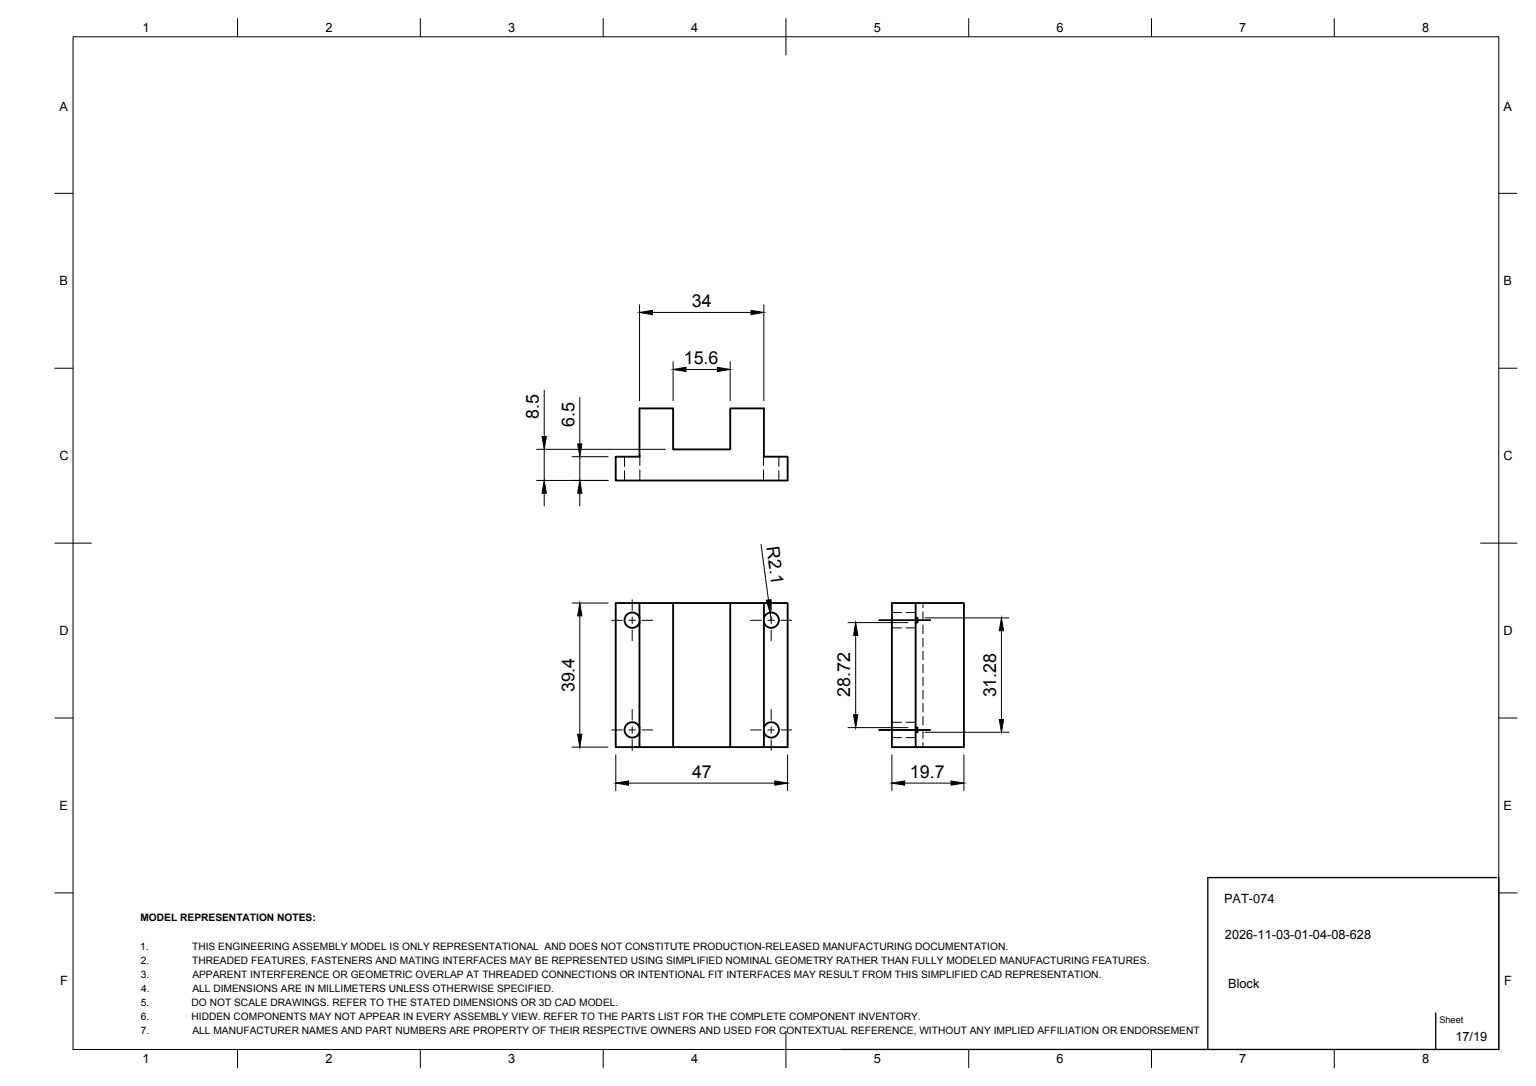
ISO-10303-21;
HEADER;
/* Generated by software containing ST-Developer
 * from STEP Tools, Inc. (www.steptools.com) 
 */

FILE_DESCRIPTION(
/* description */ ('Manual rail carriage with stops'),
/* implementation_level */ '2;1');

FILE_NAME(
/* name */ 'Block.step',
/* time_stamp */ '2026-10-27T18:54:27-07:00',
/* author */ (''),
/* organization */ (''),
/* preprocessor_version */ 'ST-DEVELOPER v20.2',
/* originating_system */ 'Autodesk Translation Framework v15.17.0.0',
/* authorisation */ '');

FILE_SCHEMA (('AUTOMOTIVE_DESIGN { 1 0 10303 214 3 1 1 }'));
ENDSEC;

DATA;
#10=MECHANICAL_DESIGN_GEOMETRIC_PRESENTATION_REPRESENTATION('',(#282),#8499);
#246=SHAPE_REPRESENTATION_RELATIONSHIP('SRR','None',#8611,#264);
#264=ADVANCED_BREP_SHAPE_REPRESENTATION('',(#298),#8490);
#282=STYLED_ITEM('',(#8767),#298);
#298=MANIFOLD_SOLID_BREP('Body1',#4952);
#356=FACE_BOUND('',#1071,.T.);
#357=FACE_BOUND('',#1072,.T.);
#358=FACE_BOUND('',#1073,.T.);
#359=FACE_BOUND('',#1074,.T.);
#505=PLANE('',#5415);
#506=PLANE('',#5421);
#507=PLANE('',#5427);
#508=PLANE('',#5433);
#509=PLANE('',#5439);
#510=PLANE('',#5440);
#511=PLANE('',#5441);
#512=PLANE('',#5442);
#513=PLANE('',#5443);
#514=PLANE('',#5444);
#515=PLANE('',#5445);
#516=PLANE('',#5446);
#517=PLANE('',#5447);
#518=PLANE('',#5448);
#519=PLANE('',#5449);
#520=PLANE('',#5450);
#521=PLANE('',#5451);
#522=PLANE('',#5452);
#741=FACE_OUTER_BOUND('',#1057,.T.);
#742=FACE_OUTER_BOUND('',#1058,.T.);
#743=FACE_OUTER_BOUND('',#1059,.T.);
#744=FACE_OUTER_BOUND('',#1060,.T.);
#745=FACE_OUTER_BOUND('',#1061,.T.);
#746=FACE_OUTER_BOUND('',#1062,.T.);
#747=FACE_OUTER_BOUND('',#1063,.T.);
#748=FACE_OUTER_BOUND('',#1064,.T.);
#749=FACE_OUTER_BOUND('',#1065,.T.);
#750=FACE_OUTER_BOUND('',#1066,.T.);
#751=FACE_OUTER_BOUND('',#1067,.T.);
#752=FACE_OUTER_BOUND('',#1068,.T.);
#753=FACE_OUTER_BOUND('',#1069,.T.);
#754=FACE_OUTER_BOUND('',#1070,.T.);
#755=FACE_OUTER_BOUND('',#1075,.T.);
#756=FACE_OUTER_BOUND('',#1076,.T.);
#757=FACE_OUTER_BOUND('',#1077,.T.);
#758=FACE_OUTER_BOUND('',#1078,.T.);
#759=FACE_OUTER_BOUND('',#1079,.T.);
#760=FACE_OUTER_BOUND('',#1080,.T.);
#761=FACE_OUTER_BOUND('',#1081,.T.);
#762=FACE_OUTER_BOUND('',#1082,.T.);
#1057=EDGE_LOOP('',(#4156,#4157));
#1058=EDGE_LOOP('',(#4158,#4159,#4160,#4161,#4162,#4163,#4164,#4165));
#1059=EDGE_LOOP('',(#4166,#4167));
#1060=EDGE_LOOP('',(#4168,#4169,#4170,#4171,#4172,#4173,#4174,#4175));
#1061=EDGE_LOOP('',(#4176,#4177));
#1062=EDGE_LOOP('',(#4178,#4179,#4180,#4181,#4182,#4183,#4184,#4185));
#1063=EDGE_LOOP('',(#4186,#4187));
#1064=EDGE_LOOP('',(#4188,#4189,#4190,#4191,#4192,#4193,#4194,#4195));
#1065=EDGE_LOOP('',(#4196,#4197,#4198,#4199,#4200,#4201,#4202,#4203,#4204,
#4205,#4206,#4207));
#1066=EDGE_LOOP('',(#4208,#4209,#4210,#4211,#4212,#4213,#4214,#4215,#4216,
#4217,#4218,#4219));
#1067=EDGE_LOOP('',(#4220,#4221,#4222,#4223,#4224,#4225,#4226,#4227,#4228,
#4229,#4230,#4231));
#1068=EDGE_LOOP('',(#4232,#4233,#4234,#4235,#4236,#4237,#4238,#4239,#4240,
#4241));
#1069=EDGE_LOOP('',(#4242,#4243,#4244,#4245));
#1070=EDGE_LOOP('',(#4246,#4247,#4248,#4249));
#1071=EDGE_LOOP('',(#4250));
#1072=EDGE_LOOP('',(#4251));
#1073=EDGE_LOOP('',(#4252));
#1074=EDGE_LOOP('',(#4253));
#1075=EDGE_LOOP('',(#4254,#4255,#4256,#4257));
#1076=EDGE_LOOP('',(#4258,#4259,#4260,#4261,#4262,#4263,#4264,#4265,#4266,
#4267));
#1077=EDGE_LOOP('',(#4268,#4269,#4270,#4271));
#1078=EDGE_LOOP('',(#4272,#4273,#4274,#4275));
#1079=EDGE_LOOP('',(#4276,#4277,#4278,#4279));
#1080=EDGE_LOOP('',(#4280,#4281,#4282,#4283));
#1081=EDGE_LOOP('',(#4284,#4285,#4286,#4287));
#1082=EDGE_LOOP('',(#4288,#4289,#4290,#4291,#4292,#4293,#4294,#4295,#4296,
#4297,#4298,#4299));
#1505=LINE('',#7911,#2005);
#1506=LINE('',#7915,#2006);
#1507=LINE('',#7919,#2007);
#1508=LINE('',#7923,#2008);
#1509=LINE('',#7927,#2009);
#1510=LINE('',#7931,#2010);
#1511=LINE('',#7935,#2011);
#1512=LINE('',#7939,#2012);
#1513=LINE('',#7943,#2013);
#1514=LINE('',#7947,#2014);
#1515=LINE('',#7951,#2015);
#1516=LINE('',#7955,#2016);
#1517=LINE('',#7959,#2017);
#1518=LINE('',#7963,#2018);
#1519=LINE('',#7967,#2019);
#1520=LINE('',#7971,#2020);
#1521=LINE('',#7973,#2021);
#1522=LINE('',#7975,#2022);
#1523=LINE('',#7977,#2023);
#1524=LINE('',#7979,#2024);
#1525=LINE('',#7981,#2025);
#1526=LINE('',#7982,#2026);
#1527=LINE('',#7984,#2027);
#1528=LINE('',#7986,#2028);
#1529=LINE('',#7988,#2029);
#1530=LINE('',#7990,#2030);
#1531=LINE('',#7992,#2031);
#1532=LINE('',#7993,#2032);
#1533=LINE('',#7996,#2033);
#1534=LINE('',#7998,#2034);
#1535=LINE('',#8000,#2035);
#1536=LINE('',#8002,#2036);
#1537=LINE('',#8003,#2037);
#1538=LINE('',#8005,#2038);
#1539=LINE('',#8007,#2039);
#1540=LINE('',#8009,#2040);
#1541=LINE('',#8011,#2041);
#1542=LINE('',#8012,#2042);
#1543=LINE('',#8015,#2043);
#1544=LINE('',#8016,#2044);
#1545=LINE('',#8019,#2045);
#1546=LINE('',#8020,#2046);
#1547=LINE('',#8023,#2047);
#1548=LINE('',#8024,#2048);
#1549=LINE('',#8027,#2049);
#1550=LINE('',#8028,#2050);
#1551=LINE('',#8030,#2051);
#1552=LINE('',#8033,#2052);
#1553=LINE('',#8034,#2053);
#1554=LINE('',#8037,#2054);
#1555=LINE('',#8038,#2055);
#1556=LINE('',#8041,#2056);
#1557=LINE('',#8042,#2057);
#1558=LINE('',#8045,#2058);
#1559=LINE('',#8046,#2059);
#1560=LINE('',#8048,#2060);
#2005=VECTOR('',#6462,1.);
#2006=VECTOR('',#6467,1.);
#2007=VECTOR('',#6470,0.21);
#2008=VECTOR('',#6475,1.);
#2009=VECTOR('',#6478,1.);
#2010=VECTOR('',#6483,1.);
#2011=VECTOR('',#6486,0.21);
#2012=VECTOR('',#6491,1.);
#2013=VECTOR('',#6494,1.);
#2014=VECTOR('',#6499,1.);
#2015=VECTOR('',#6502,0.21);
#2016=VECTOR('',#6507,1.);
#2017=VECTOR('',#6510,1.);
#2018=VECTOR('',#6515,1.);
#2019=VECTOR('',#6518,0.21);
#2020=VECTOR('',#6523,1.);
#2021=VECTOR('',#6526,1.);
#2022=VECTOR('',#6527,1.);
#2023=VECTOR('',#6528,1.);
#2024=VECTOR('',#6529,1.);
#2025=VECTOR('',#6530,1.);
#2026=VECTOR('',#6531,1.);
#2027=VECTOR('',#6534,1.);
#2028=VECTOR('',#6535,1.);
#2029=VECTOR('',#6536,1.);
#2030=VECTOR('',#6537,1.);
#2031=VECTOR('',#6538,1.);
#2032=VECTOR('',#6539,1.);
#2033=VECTOR('',#6542,1.);
#2034=VECTOR('',#6543,1.);
#2035=VECTOR('',#6544,1.);
#2036=VECTOR('',#6545,1.);
#2037=VECTOR('',#6546,1.);
#2038=VECTOR('',#6547,1.);
#2039=VECTOR('',#6548,1.);
#2040=VECTOR('',#6549,1.);
#2041=VECTOR('',#6550,1.);
#2042=VECTOR('',#6551,1.);
#2043=VECTOR('',#6554,1.);
#2044=VECTOR('',#6555,1.);
#2045=VECTOR('',#6558,1.);
#2046=VECTOR('',#6559,1.);
#2047=VECTOR('',#6562,1.);
#2048=VECTOR('',#6563,1.);
#2049=VECTOR('',#6566,1.);
#2050=VECTOR('',#6567,1.);
#2051=VECTOR('',#6570,1.);
#2052=VECTOR('',#6573,1.);
#2053=VECTOR('',#6574,1.);
#2054=VECTOR('',#6577,1.);
#2055=VECTOR('',#6578,1.);
#2056=VECTOR('',#6581,1.);
#2057=VECTOR('',#6582,1.);
#2058=VECTOR('',#6585,1.);
#2059=VECTOR('',#6586,1.);
#2060=VECTOR('',#6589,1.);
#2255=CIRCLE('',#5416,0.21);
#2256=CIRCLE('',#5418,0.21);
#2257=CIRCLE('',#5419,0.21);
#2258=CIRCLE('',#5420,0.21);
#2259=CIRCLE('',#5422,0.21);
#2260=CIRCLE('',#5424,0.21);
#2261=CIRCLE('',#5425,0.21);
#2262=CIRCLE('',#5426,0.21);
#2263=CIRCLE('',#5428,0.21);
#2264=CIRCLE('',#5430,0.21);
#2265=CIRCLE('',#5431,0.21);
#2266=CIRCLE('',#5432,0.21);
#2267=CIRCLE('',#5434,0.21);
#2268=CIRCLE('',#5436,0.21);
#2269=CIRCLE('',#5437,0.21);
#2270=CIRCLE('',#5438,0.21);
#2575=VERTEX_POINT('',#7909);
#2576=VERTEX_POINT('',#7910);
#2577=VERTEX_POINT('',#7914);
#2578=VERTEX_POINT('',#7916);
#2579=VERTEX_POINT('',#7918);
#2580=VERTEX_POINT('',#7921);
#2581=VERTEX_POINT('',#7925);
#2582=VERTEX_POINT('',#7926);
#2583=VERTEX_POINT('',#7930);
#2584=VERTEX_POINT('',#7932);
#2585=VERTEX_POINT('',#7934);
#2586=VERTEX_POINT('',#7937);
#2587=VERTEX_POINT('',#7941);
#2588=VERTEX_POINT('',#7942);
#2589=VERTEX_POINT('',#7946);
#2590=VERTEX_POINT('',#7948);
#2591=VERTEX_POINT('',#7950);
#2592=VERTEX_POINT('',#7953);
#2593=VERTEX_POINT('',#7957);
#2594=VERTEX_POINT('',#7958);
#2595=VERTEX_POINT('',#7962);
#2596=VERTEX_POINT('',#7964);
#2597=VERTEX_POINT('',#7966);
#2598=VERTEX_POINT('',#7969);
#2599=VERTEX_POINT('',#7974);
#2600=VERTEX_POINT('',#7976);
#2601=VERTEX_POINT('',#7978);
#2602=VERTEX_POINT('',#7980);
#2603=VERTEX_POINT('',#7985);
#2604=VERTEX_POINT('',#7987);
#2605=VERTEX_POINT('',#7989);
#2606=VERTEX_POINT('',#7991);
#2607=VERTEX_POINT('',#7995);
#2608=VERTEX_POINT('',#7997);
#2609=VERTEX_POINT('',#7999);
#2610=VERTEX_POINT('',#8001);
#2611=VERTEX_POINT('',#8004);
#2612=VERTEX_POINT('',#8006);
#2613=VERTEX_POINT('',#8008);
#2614=VERTEX_POINT('',#8010);
#2615=VERTEX_POINT('',#8014);
#2616=VERTEX_POINT('',#8018);
#2617=VERTEX_POINT('',#8022);
#2618=VERTEX_POINT('',#8026);
#2619=VERTEX_POINT('',#8032);
#2620=VERTEX_POINT('',#8036);
#2621=VERTEX_POINT('',#8040);
#2622=VERTEX_POINT('',#8044);
#3126=EDGE_CURVE('',#2575,#2576,#1505,.T.);
#3127=EDGE_CURVE('',#2575,#2576,#2255,.T.);
#3128=EDGE_CURVE('',#2577,#2575,#1506,.T.);
#3129=EDGE_CURVE('',#2578,#2577,#2256,.T.);
#3130=EDGE_CURVE('',#2578,#2579,#1507,.T.);
#3131=EDGE_CURVE('',#2579,#2579,#2257,.T.);
#3132=EDGE_CURVE('',#2580,#2578,#2258,.T.);
#3133=EDGE_CURVE('',#2576,#2580,#1508,.T.);
#3134=EDGE_CURVE('',#2581,#2582,#1509,.T.);
#3135=EDGE_CURVE('',#2581,#2582,#2259,.T.);
#3136=EDGE_CURVE('',#2583,#2581,#1510,.T.);
#3137=EDGE_CURVE('',#2584,#2583,#2260,.T.);
#3138=EDGE_CURVE('',#2584,#2585,#1511,.T.);
#3139=EDGE_CURVE('',#2585,#2585,#2261,.T.);
#3140=EDGE_CURVE('',#2586,#2584,#2262,.T.);
#3141=EDGE_CURVE('',#2582,#2586,#1512,.T.);
#3142=EDGE_CURVE('',#2587,#2588,#1513,.T.);
#3143=EDGE_CURVE('',#2587,#2588,#2263,.T.);
#3144=EDGE_CURVE('',#2589,#2587,#1514,.T.);
#3145=EDGE_CURVE('',#2590,#2589,#2264,.T.);
#3146=EDGE_CURVE('',#2590,#2591,#1515,.T.);
#3147=EDGE_CURVE('',#2591,#2591,#2265,.T.);
#3148=EDGE_CURVE('',#2592,#2590,#2266,.T.);
#3149=EDGE_CURVE('',#2588,#2592,#1516,.T.);
#3150=EDGE_CURVE('',#2593,#2594,#1517,.T.);
#3151=EDGE_CURVE('',#2593,#2594,#2267,.T.);
#3152=EDGE_CURVE('',#2595,#2593,#1518,.T.);
#3153=EDGE_CURVE('',#2596,#2595,#2268,.T.);
#3154=EDGE_CURVE('',#2596,#2597,#1519,.T.);
#3155=EDGE_CURVE('',#2597,#2597,#2269,.T.);
#3156=EDGE_CURVE('',#2598,#2596,#2270,.T.);
#3157=EDGE_CURVE('',#2594,#2598,#1520,.T.);
#3158=EDGE_CURVE('',#2580,#2589,#1521,.T.);
#3159=EDGE_CURVE('',#2592,#2599,#1522,.T.);
#3160=EDGE_CURVE('',#2600,#2599,#1523,.T.);
#3161=EDGE_CURVE('',#2600,#2601,#1524,.T.);
#3162=EDGE_CURVE('',#2602,#2601,#1525,.T.);
#3163=EDGE_CURVE('',#2602,#2577,#1526,.T.);
#3164=EDGE_CURVE('',#2586,#2595,#1527,.T.);
#3165=EDGE_CURVE('',#2598,#2603,#1528,.T.);
#3166=EDGE_CURVE('',#2604,#2603,#1529,.T.);
#3167=EDGE_CURVE('',#2605,#2604,#1530,.T.);
#3168=EDGE_CURVE('',#2606,#2605,#1531,.T.);
#3169=EDGE_CURVE('',#2606,#2583,#1532,.T.);
#3170=EDGE_CURVE('',#2599,#2607,#1533,.T.);
#3171=EDGE_CURVE('',#2607,#2608,#1534,.T.);
#3172=EDGE_CURVE('',#2608,#2609,#1535,.T.);
#3173=EDGE_CURVE('',#2609,#2610,#1536,.T.);
#3174=EDGE_CURVE('',#2610,#2606,#1537,.T.);
#3175=EDGE_CURVE('',#2605,#2611,#1538,.T.);
#3176=EDGE_CURVE('',#2611,#2612,#1539,.T.);
#3177=EDGE_CURVE('',#2612,#2613,#1540,.T.);
#3178=EDGE_CURVE('',#2613,#2614,#1541,.T.);
#3179=EDGE_CURVE('',#2614,#2600,#1542,.T.);
#3180=EDGE_CURVE('',#2615,#2602,#1543,.T.);
#3181=EDGE_CURVE('',#2607,#2615,#1544,.T.);
#3182=EDGE_CURVE('',#2616,#2615,#1545,.T.);
#3183=EDGE_CURVE('',#2608,#2616,#1546,.T.);
#3184=EDGE_CURVE('',#2617,#2616,#1547,.T.);
#3185=EDGE_CURVE('',#2609,#2617,#1548,.T.);
#3186=EDGE_CURVE('',#2618,#2617,#1549,.T.);
#3187=EDGE_CURVE('',#2610,#2618,#1550,.T.);
#3188=EDGE_CURVE('',#2603,#2618,#1551,.T.);
#3189=EDGE_CURVE('',#2619,#2604,#1552,.T.);
#3190=EDGE_CURVE('',#2611,#2619,#1553,.T.);
#3191=EDGE_CURVE('',#2620,#2619,#1554,.T.);
#3192=EDGE_CURVE('',#2612,#2620,#1555,.T.);
#3193=EDGE_CURVE('',#2621,#2620,#1556,.T.);
#3194=EDGE_CURVE('',#2613,#2621,#1557,.T.);
#3195=EDGE_CURVE('',#2622,#2621,#1558,.T.);
#3196=EDGE_CURVE('',#2614,#2622,#1559,.T.);
#3197=EDGE_CURVE('',#2601,#2622,#1560,.T.);
#4156=ORIENTED_EDGE('',*,*,#3126,.F.);
#4157=ORIENTED_EDGE('',*,*,#3127,.T.);
#4158=ORIENTED_EDGE('',*,*,#3128,.F.);
#4159=ORIENTED_EDGE('',*,*,#3129,.F.);
#4160=ORIENTED_EDGE('',*,*,#3130,.T.);
#4161=ORIENTED_EDGE('',*,*,#3131,.F.);
#4162=ORIENTED_EDGE('',*,*,#3130,.F.);
#4163=ORIENTED_EDGE('',*,*,#3132,.F.);
#4164=ORIENTED_EDGE('',*,*,#3133,.F.);
#4165=ORIENTED_EDGE('',*,*,#3127,.F.);
#4166=ORIENTED_EDGE('',*,*,#3134,.F.);
#4167=ORIENTED_EDGE('',*,*,#3135,.T.);
#4168=ORIENTED_EDGE('',*,*,#3136,.F.);
#4169=ORIENTED_EDGE('',*,*,#3137,.F.);
#4170=ORIENTED_EDGE('',*,*,#3138,.T.);
#4171=ORIENTED_EDGE('',*,*,#3139,.F.);
#4172=ORIENTED_EDGE('',*,*,#3138,.F.);
#4173=ORIENTED_EDGE('',*,*,#3140,.F.);
#4174=ORIENTED_EDGE('',*,*,#3141,.F.);
#4175=ORIENTED_EDGE('',*,*,#3135,.F.);
#4176=ORIENTED_EDGE('',*,*,#3142,.F.);
#4177=ORIENTED_EDGE('',*,*,#3143,.T.);
#4178=ORIENTED_EDGE('',*,*,#3144,.F.);
#4179=ORIENTED_EDGE('',*,*,#3145,.F.);
#4180=ORIENTED_EDGE('',*,*,#3146,.T.);
#4181=ORIENTED_EDGE('',*,*,#3147,.F.);
#4182=ORIENTED_EDGE('',*,*,#3146,.F.);
#4183=ORIENTED_EDGE('',*,*,#3148,.F.);
#4184=ORIENTED_EDGE('',*,*,#3149,.F.);
#4185=ORIENTED_EDGE('',*,*,#3143,.F.);
#4186=ORIENTED_EDGE('',*,*,#3150,.F.);
#4187=ORIENTED_EDGE('',*,*,#3151,.T.);
#4188=ORIENTED_EDGE('',*,*,#3152,.F.);
#4189=ORIENTED_EDGE('',*,*,#3153,.F.);
#4190=ORIENTED_EDGE('',*,*,#3154,.T.);
#4191=ORIENTED_EDGE('',*,*,#3155,.F.);
#4192=ORIENTED_EDGE('',*,*,#3154,.F.);
#4193=ORIENTED_EDGE('',*,*,#3156,.F.);
#4194=ORIENTED_EDGE('',*,*,#3157,.F.);
#4195=ORIENTED_EDGE('',*,*,#3151,.F.);
#4196=ORIENTED_EDGE('',*,*,#3128,.T.);
#4197=ORIENTED_EDGE('',*,*,#3126,.T.);
#4198=ORIENTED_EDGE('',*,*,#3133,.T.);
#4199=ORIENTED_EDGE('',*,*,#3158,.T.);
#4200=ORIENTED_EDGE('',*,*,#3144,.T.);
#4201=ORIENTED_EDGE('',*,*,#3142,.T.);
#4202=ORIENTED_EDGE('',*,*,#3149,.T.);
#4203=ORIENTED_EDGE('',*,*,#3159,.T.);
#4204=ORIENTED_EDGE('',*,*,#3160,.F.);
#4205=ORIENTED_EDGE('',*,*,#3161,.T.);
#4206=ORIENTED_EDGE('',*,*,#3162,.F.);
#4207=ORIENTED_EDGE('',*,*,#3163,.T.);
#4208=ORIENTED_EDGE('',*,*,#3136,.T.);
#4209=ORIENTED_EDGE('',*,*,#3134,.T.);
#4210=ORIENTED_EDGE('',*,*,#3141,.T.);
#4211=ORIENTED_EDGE('',*,*,#3164,.T.);
#4212=ORIENTED_EDGE('',*,*,#3152,.T.);
#4213=ORIENTED_EDGE('',*,*,#3150,.T.);
#4214=ORIENTED_EDGE('',*,*,#3157,.T.);
#4215=ORIENTED_EDGE('',*,*,#3165,.T.);
#4216=ORIENTED_EDGE('',*,*,#3166,.F.);
#4217=ORIENTED_EDGE('',*,*,#3167,.F.);
#4218=ORIENTED_EDGE('',*,*,#3168,.F.);
#4219=ORIENTED_EDGE('',*,*,#3169,.T.);
#4220=ORIENTED_EDGE('',*,*,#3160,.T.);
#4221=ORIENTED_EDGE('',*,*,#3170,.T.);
#4222=ORIENTED_EDGE('',*,*,#3171,.T.);
#4223=ORIENTED_EDGE('',*,*,#3172,.T.);
#4224=ORIENTED_EDGE('',*,*,#3173,.T.);
#4225=ORIENTED_EDGE('',*,*,#3174,.T.);
#4226=ORIENTED_EDGE('',*,*,#3168,.T.);
#4227=ORIENTED_EDGE('',*,*,#3175,.T.);
#4228=ORIENTED_EDGE('',*,*,#3176,.T.);
#4229=ORIENTED_EDGE('',*,*,#3177,.T.);
#4230=ORIENTED_EDGE('',*,*,#3178,.T.);
#4231=ORIENTED_EDGE('',*,*,#3179,.T.);
#4232=ORIENTED_EDGE('',*,*,#3132,.T.);
#4233=ORIENTED_EDGE('',*,*,#3129,.T.);
#4234=ORIENTED_EDGE('',*,*,#3163,.F.);
#4235=ORIENTED_EDGE('',*,*,#3180,.F.);
#4236=ORIENTED_EDGE('',*,*,#3181,.F.);
#4237=ORIENTED_EDGE('',*,*,#3170,.F.);
#4238=ORIENTED_EDGE('',*,*,#3159,.F.);
#4239=ORIENTED_EDGE('',*,*,#3148,.T.);
#4240=ORIENTED_EDGE('',*,*,#3145,.T.);
#4241=ORIENTED_EDGE('',*,*,#3158,.F.);
#4242=ORIENTED_EDGE('',*,*,#3181,.T.);
#4243=ORIENTED_EDGE('',*,*,#3182,.F.);
#4244=ORIENTED_EDGE('',*,*,#3183,.F.);
#4245=ORIENTED_EDGE('',*,*,#3171,.F.);
#4246=ORIENTED_EDGE('',*,*,#3183,.T.);
#4247=ORIENTED_EDGE('',*,*,#3184,.F.);
#4248=ORIENTED_EDGE('',*,*,#3185,.F.);
#4249=ORIENTED_EDGE('',*,*,#3172,.F.);
#4250=ORIENTED_EDGE('',*,*,#3131,.T.);
#4251=ORIENTED_EDGE('',*,*,#3139,.T.);
#4252=ORIENTED_EDGE('',*,*,#3147,.T.);
#4253=ORIENTED_EDGE('',*,*,#3155,.T.);
#4254=ORIENTED_EDGE('',*,*,#3185,.T.);
#4255=ORIENTED_EDGE('',*,*,#3186,.F.);
#4256=ORIENTED_EDGE('',*,*,#3187,.F.);
#4257=ORIENTED_EDGE('',*,*,#3173,.F.);
#4258=ORIENTED_EDGE('',*,*,#3140,.T.);
#4259=ORIENTED_EDGE('',*,*,#3137,.T.);
#4260=ORIENTED_EDGE('',*,*,#3169,.F.);
#4261=ORIENTED_EDGE('',*,*,#3174,.F.);
#4262=ORIENTED_EDGE('',*,*,#3187,.T.);
#4263=ORIENTED_EDGE('',*,*,#3188,.F.);
#4264=ORIENTED_EDGE('',*,*,#3165,.F.);
#4265=ORIENTED_EDGE('',*,*,#3156,.T.);
#4266=ORIENTED_EDGE('',*,*,#3153,.T.);
#4267=ORIENTED_EDGE('',*,*,#3164,.F.);
#4268=ORIENTED_EDGE('',*,*,#3167,.T.);
#4269=ORIENTED_EDGE('',*,*,#3189,.F.);
#4270=ORIENTED_EDGE('',*,*,#3190,.F.);
#4271=ORIENTED_EDGE('',*,*,#3175,.F.);
#4272=ORIENTED_EDGE('',*,*,#3190,.T.);
#4273=ORIENTED_EDGE('',*,*,#3191,.F.);
#4274=ORIENTED_EDGE('',*,*,#3192,.F.);
#4275=ORIENTED_EDGE('',*,*,#3176,.F.);
#4276=ORIENTED_EDGE('',*,*,#3192,.T.);
#4277=ORIENTED_EDGE('',*,*,#3193,.F.);
#4278=ORIENTED_EDGE('',*,*,#3194,.F.);
#4279=ORIENTED_EDGE('',*,*,#3177,.F.);
#4280=ORIENTED_EDGE('',*,*,#3194,.T.);
#4281=ORIENTED_EDGE('',*,*,#3195,.F.);
#4282=ORIENTED_EDGE('',*,*,#3196,.F.);
#4283=ORIENTED_EDGE('',*,*,#3178,.F.);
#4284=ORIENTED_EDGE('',*,*,#3196,.T.);
#4285=ORIENTED_EDGE('',*,*,#3197,.F.);
#4286=ORIENTED_EDGE('',*,*,#3161,.F.);
#4287=ORIENTED_EDGE('',*,*,#3179,.F.);
#4288=ORIENTED_EDGE('',*,*,#3162,.T.);
#4289=ORIENTED_EDGE('',*,*,#3197,.T.);
#4290=ORIENTED_EDGE('',*,*,#3195,.T.);
#4291=ORIENTED_EDGE('',*,*,#3193,.T.);
#4292=ORIENTED_EDGE('',*,*,#3191,.T.);
#4293=ORIENTED_EDGE('',*,*,#3189,.T.);
#4294=ORIENTED_EDGE('',*,*,#3166,.T.);
#4295=ORIENTED_EDGE('',*,*,#3188,.T.);
#4296=ORIENTED_EDGE('',*,*,#3186,.T.);
#4297=ORIENTED_EDGE('',*,*,#3184,.T.);
#4298=ORIENTED_EDGE('',*,*,#3182,.T.);
#4299=ORIENTED_EDGE('',*,*,#3180,.T.);
#4656=CYLINDRICAL_SURFACE('',#5417,0.21);
#4657=CYLINDRICAL_SURFACE('',#5423,0.21);
#4658=CYLINDRICAL_SURFACE('',#5429,0.21);
#4659=CYLINDRICAL_SURFACE('',#5435,0.21);
#4840=ADVANCED_FACE('',(#741),#505,.T.);
#4841=ADVANCED_FACE('',(#742),#4656,.F.);
#4842=ADVANCED_FACE('',(#743),#506,.T.);
#4843=ADVANCED_FACE('',(#744),#4657,.F.);
#4844=ADVANCED_FACE('',(#745),#507,.T.);
#4845=ADVANCED_FACE('',(#746),#4658,.F.);
#4846=ADVANCED_FACE('',(#747),#508,.T.);
#4847=ADVANCED_FACE('',(#748),#4659,.F.);
#4848=ADVANCED_FACE('',(#749),#509,.T.);
#4849=ADVANCED_FACE('',(#750),#510,.T.);
#4850=ADVANCED_FACE('',(#751),#511,.T.);
#4851=ADVANCED_FACE('',(#752),#512,.T.);
#4852=ADVANCED_FACE('',(#753),#513,.T.);
#4853=ADVANCED_FACE('',(#754,#356,#357,#358,#359),#514,.T.);
#4854=ADVANCED_FACE('',(#755),#515,.T.);
#4855=ADVANCED_FACE('',(#756),#516,.T.);
#4856=ADVANCED_FACE('',(#757),#517,.T.);
#4857=ADVANCED_FACE('',(#758),#518,.T.);
#4858=ADVANCED_FACE('',(#759),#519,.T.);
#4859=ADVANCED_FACE('',(#760),#520,.T.);
#4860=ADVANCED_FACE('',(#761),#521,.T.);
#4861=ADVANCED_FACE('',(#762),#522,.T.);
#4952=CLOSED_SHELL('',(#4840,#4841,#4842,#4843,#4844,#4845,#4846,#4847,
#4848,#4849,#4850,#4851,#4852,#4853,#4854,#4855,#4856,#4857,#4858,#4859,
#4860,#4861));
#5414=AXIS2_PLACEMENT_3D('',#7907,#6458,#6459);
#5415=AXIS2_PLACEMENT_3D('',#7908,#6460,#6461);
#5416=AXIS2_PLACEMENT_3D('',#7912,#6463,#6464);
#5417=AXIS2_PLACEMENT_3D('',#7913,#6465,#6466);
#5418=AXIS2_PLACEMENT_3D('',#7917,#6468,#6469);
#5419=AXIS2_PLACEMENT_3D('',#7920,#6471,#6472);
#5420=AXIS2_PLACEMENT_3D('',#7922,#6473,#6474);
#5421=AXIS2_PLACEMENT_3D('',#7924,#6476,#6477);
#5422=AXIS2_PLACEMENT_3D('',#7928,#6479,#6480);
#5423=AXIS2_PLACEMENT_3D('',#7929,#6481,#6482);
#5424=AXIS2_PLACEMENT_3D('',#7933,#6484,#6485);
#5425=AXIS2_PLACEMENT_3D('',#7936,#6487,#6488);
#5426=AXIS2_PLACEMENT_3D('',#7938,#6489,#6490);
#5427=AXIS2_PLACEMENT_3D('',#7940,#6492,#6493);
#5428=AXIS2_PLACEMENT_3D('',#7944,#6495,#6496);
#5429=AXIS2_PLACEMENT_3D('',#7945,#6497,#6498);
#5430=AXIS2_PLACEMENT_3D('',#7949,#6500,#6501);
#5431=AXIS2_PLACEMENT_3D('',#7952,#6503,#6504);
#5432=AXIS2_PLACEMENT_3D('',#7954,#6505,#6506);
#5433=AXIS2_PLACEMENT_3D('',#7956,#6508,#6509);
#5434=AXIS2_PLACEMENT_3D('',#7960,#6511,#6512);
#5435=AXIS2_PLACEMENT_3D('',#7961,#6513,#6514);
#5436=AXIS2_PLACEMENT_3D('',#7965,#6516,#6517);
#5437=AXIS2_PLACEMENT_3D('',#7968,#6519,#6520);
#5438=AXIS2_PLACEMENT_3D('',#7970,#6521,#6522);
#5439=AXIS2_PLACEMENT_3D('',#7972,#6524,#6525);
#5440=AXIS2_PLACEMENT_3D('',#7983,#6532,#6533);
#5441=AXIS2_PLACEMENT_3D('',#7994,#6540,#6541);
#5442=AXIS2_PLACEMENT_3D('',#8013,#6552,#6553);
#5443=AXIS2_PLACEMENT_3D('',#8017,#6556,#6557);
#5444=AXIS2_PLACEMENT_3D('',#8021,#6560,#6561);
#5445=AXIS2_PLACEMENT_3D('',#8025,#6564,#6565);
#5446=AXIS2_PLACEMENT_3D('',#8029,#6568,#6569);
#5447=AXIS2_PLACEMENT_3D('',#8031,#6571,#6572);
#5448=AXIS2_PLACEMENT_3D('',#8035,#6575,#6576);
#5449=AXIS2_PLACEMENT_3D('',#8039,#6579,#6580);
#5450=AXIS2_PLACEMENT_3D('',#8043,#6583,#6584);
#5451=AXIS2_PLACEMENT_3D('',#8047,#6587,#6588);
#5452=AXIS2_PLACEMENT_3D('',#8049,#6590,#6591);
#6458=DIRECTION('axis',(0.,0.,1.));
#6459=DIRECTION('refdir',(1.,0.,0.));
#6460=DIRECTION('center_axis',(0.,0.,1.));
#6461=DIRECTION('ref_axis',(1.,0.,0.));
#6462=DIRECTION('',(-1.,0.,0.));
#6463=DIRECTION('center_axis',(0.,0.,1.));
#6464=DIRECTION('ref_axis',(1.,0.,0.));
#6465=DIRECTION('center_axis',(0.,0.,1.));
#6466=DIRECTION('ref_axis',(1.,0.,0.));
#6467=DIRECTION('',(0.,0.,-1.));
#6468=DIRECTION('center_axis',(0.,0.,1.));
#6469=DIRECTION('ref_axis',(1.,0.,0.));
#6470=DIRECTION('',(0.,0.,1.));
#6471=DIRECTION('center_axis',(0.,0.,-1.));
#6472=DIRECTION('ref_axis',(1.,0.,0.));
#6473=DIRECTION('center_axis',(0.,0.,1.));
#6474=DIRECTION('ref_axis',(1.,0.,0.));
#6475=DIRECTION('',(0.,0.,1.));
#6476=DIRECTION('center_axis',(0.,0.,1.));
#6477=DIRECTION('ref_axis',(1.,0.,0.));
#6478=DIRECTION('',(1.,0.,0.));
#6479=DIRECTION('center_axis',(0.,0.,1.));
#6480=DIRECTION('ref_axis',(1.,0.,0.));
#6481=DIRECTION('center_axis',(0.,0.,1.));
#6482=DIRECTION('ref_axis',(1.,0.,0.));
#6483=DIRECTION('',(0.,0.,-1.));
#6484=DIRECTION('center_axis',(0.,0.,1.));
#6485=DIRECTION('ref_axis',(1.,0.,0.));
#6486=DIRECTION('',(0.,0.,1.));
#6487=DIRECTION('center_axis',(0.,0.,-1.));
#6488=DIRECTION('ref_axis',(1.,0.,0.));
#6489=DIRECTION('center_axis',(0.,0.,1.));
#6490=DIRECTION('ref_axis',(1.,0.,0.));
#6491=DIRECTION('',(0.,0.,1.));
#6492=DIRECTION('center_axis',(0.,0.,1.));
#6493=DIRECTION('ref_axis',(1.,0.,0.));
#6494=DIRECTION('',(-1.,0.,0.));
#6495=DIRECTION('center_axis',(0.,0.,1.));
#6496=DIRECTION('ref_axis',(1.,0.,0.));
#6497=DIRECTION('center_axis',(0.,0.,1.));
#6498=DIRECTION('ref_axis',(1.,0.,0.));
#6499=DIRECTION('',(0.,0.,-1.));
#6500=DIRECTION('center_axis',(0.,0.,1.));
#6501=DIRECTION('ref_axis',(1.,0.,0.));
#6502=DIRECTION('',(0.,0.,1.));
#6503=DIRECTION('center_axis',(0.,0.,-1.));
#6504=DIRECTION('ref_axis',(1.,0.,0.));
#6505=DIRECTION('center_axis',(0.,0.,1.));
#6506=DIRECTION('ref_axis',(1.,0.,0.));
#6507=DIRECTION('',(0.,0.,1.));
#6508=DIRECTION('center_axis',(0.,0.,1.));
#6509=DIRECTION('ref_axis',(1.,0.,0.));
#6510=DIRECTION('',(1.,0.,0.));
#6511=DIRECTION('center_axis',(0.,0.,1.));
#6512=DIRECTION('ref_axis',(1.,0.,0.));
#6513=DIRECTION('center_axis',(0.,0.,1.));
#6514=DIRECTION('ref_axis',(1.,0.,0.));
#6515=DIRECTION('',(0.,0.,-1.));
#6516=DIRECTION('center_axis',(0.,0.,1.));
#6517=DIRECTION('ref_axis',(1.,0.,0.));
#6518=DIRECTION('',(0.,0.,1.));
#6519=DIRECTION('center_axis',(0.,0.,-1.));
#6520=DIRECTION('ref_axis',(1.,0.,0.));
#6521=DIRECTION('center_axis',(0.,0.,1.));
#6522=DIRECTION('ref_axis',(1.,0.,0.));
#6523=DIRECTION('',(0.,0.,1.));
#6524=DIRECTION('center_axis',(0.,-1.,0.));
#6525=DIRECTION('ref_axis',(0.,0.,-1.));
#6526=DIRECTION('',(-1.,0.,0.));
#6527=DIRECTION('',(-1.,0.,0.));
#6528=DIRECTION('',(0.,0.,1.));
#6529=DIRECTION('',(1.,0.,0.));
#6530=DIRECTION('',(0.,0.,-1.));
#6531=DIRECTION('',(-1.,0.,0.));
#6532=DIRECTION('center_axis',(0.,1.,0.));
#6533=DIRECTION('ref_axis',(0.,0.,1.));
#6534=DIRECTION('',(1.,0.,0.));
#6535=DIRECTION('',(1.,0.,0.));
#6536=DIRECTION('',(0.,0.,1.));
#6537=DIRECTION('',(1.,0.,0.));
#6538=DIRECTION('',(0.,0.,-1.));
#6539=DIRECTION('',(1.,0.,0.));
#6540=DIRECTION('center_axis',(-1.,0.,0.));
#6541=DIRECTION('ref_axis',(0.,0.,1.));
#6542=DIRECTION('',(0.,-1.,0.));
#6543=DIRECTION('',(0.,0.,1.));
#6544=DIRECTION('',(0.,1.,0.));
#6545=DIRECTION('',(0.,0.,-1.));
#6546=DIRECTION('',(0.,-1.,0.));
#6547=DIRECTION('',(0.,-1.,0.));
#6548=DIRECTION('',(0.,0.,1.));
#6549=DIRECTION('',(0.,-1.,0.));
#6550=DIRECTION('',(0.,0.,-1.));
#6551=DIRECTION('',(0.,-1.,0.));
#6552=DIRECTION('center_axis',(0.,0.,-1.));
#6553=DIRECTION('ref_axis',(0.,1.,0.));
#6554=DIRECTION('',(0.,1.,0.));
#6555=DIRECTION('',(1.,0.,0.));
#6556=DIRECTION('center_axis',(0.,-1.,0.));
#6557=DIRECTION('ref_axis',(0.,0.,-1.));
#6558=DIRECTION('',(0.,0.,-1.));
#6559=DIRECTION('',(1.,0.,0.));
#6560=DIRECTION('center_axis',(0.,0.,1.));
#6561=DIRECTION('ref_axis',(0.,-1.,0.));
#6562=DIRECTION('',(0.,-1.,0.));
#6563=DIRECTION('',(1.,0.,0.));
#6564=DIRECTION('center_axis',(0.,1.,0.));
#6565=DIRECTION('ref_axis',(0.,0.,1.));
#6566=DIRECTION('',(0.,0.,1.));
#6567=DIRECTION('',(1.,0.,0.));
#6568=DIRECTION('center_axis',(0.,0.,-1.));
#6569=DIRECTION('ref_axis',(0.,1.,0.));
#6570=DIRECTION('',(0.,1.,0.));
#6571=DIRECTION('center_axis',(0.,0.,-1.));
#6572=DIRECTION('ref_axis',(0.,1.,0.));
#6573=DIRECTION('',(0.,1.,0.));
#6574=DIRECTION('',(1.,0.,0.));
#6575=DIRECTION('center_axis',(0.,-1.,0.));
#6576=DIRECTION('ref_axis',(0.,0.,-1.));
#6577=DIRECTION('',(0.,0.,-1.));
#6578=DIRECTION('',(1.,0.,0.));
#6579=DIRECTION('center_axis',(0.,0.,-1.));
#6580=DIRECTION('ref_axis',(0.,1.,0.));
#6581=DIRECTION('',(0.,1.,0.));
#6582=DIRECTION('',(1.,0.,0.));
#6583=DIRECTION('center_axis',(0.,1.,0.));
#6584=DIRECTION('ref_axis',(0.,0.,1.));
#6585=DIRECTION('',(0.,0.,1.));
#6586=DIRECTION('',(1.,0.,0.));
#6587=DIRECTION('center_axis',(0.,0.,-1.));
#6588=DIRECTION('ref_axis',(0.,1.,0.));
#6589=DIRECTION('',(0.,1.,0.));
#6590=DIRECTION('center_axis',(1.,0.,0.));
#6591=DIRECTION('ref_axis',(0.,0.,-1.));
#7907=CARTESIAN_POINT('',(0.,0.,0.));
#7908=CARTESIAN_POINT('Origin',(1.5,-1.9,1.7));
#7909=CARTESIAN_POINT('',(1.56403124237433,-1.7,1.7));
#7910=CARTESIAN_POINT('',(1.43596875762567,-1.7,1.7));
#7911=CARTESIAN_POINT('',(0.75,-1.7,1.7));
#7912=CARTESIAN_POINT('Origin',(1.5,-1.9,1.7));
#7913=CARTESIAN_POINT('Origin',(1.5,-1.9,1.7));
#7914=CARTESIAN_POINT('',(1.56403124237433,-1.7,1.75));
#7915=CARTESIAN_POINT('',(1.56403124237433,-1.7,1.7));
#7916=CARTESIAN_POINT('',(1.29,-1.9,1.75));
#7917=CARTESIAN_POINT('Origin',(1.5,-1.9,1.75));
#7918=CARTESIAN_POINT('',(1.29,-1.9,2.4));
#7919=CARTESIAN_POINT('',(1.29,-1.9,1.7));
#7920=CARTESIAN_POINT('Origin',(1.5,-1.9,2.4));
#7921=CARTESIAN_POINT('',(1.43596875762567,-1.7,1.75));
#7922=CARTESIAN_POINT('Origin',(1.5,-1.9,1.75));
#7923=CARTESIAN_POINT('',(1.43596875762567,-1.7,1.7));
#7924=CARTESIAN_POINT('Origin',(-1.5,1.9,1.7));
#7925=CARTESIAN_POINT('',(-1.56403124237433,1.7,1.7));
#7926=CARTESIAN_POINT('',(-1.43596875762567,1.7,1.7));
#7927=CARTESIAN_POINT('',(-0.75,1.7,1.7));
#7928=CARTESIAN_POINT('Origin',(-1.5,1.9,1.7));
#7929=CARTESIAN_POINT('Origin',(-1.5,1.9,1.7));
#7930=CARTESIAN_POINT('',(-1.56403124237433,1.7,1.75));
#7931=CARTESIAN_POINT('',(-1.56403124237433,1.7,1.7));
#7932=CARTESIAN_POINT('',(-1.71,1.9,1.75));
#7933=CARTESIAN_POINT('Origin',(-1.5,1.9,1.75));
#7934=CARTESIAN_POINT('',(-1.71,1.9,2.4));
#7935=CARTESIAN_POINT('',(-1.71,1.9,1.7));
#7936=CARTESIAN_POINT('Origin',(-1.5,1.9,2.4));
#7937=CARTESIAN_POINT('',(-1.43596875762567,1.7,1.75));
#7938=CARTESIAN_POINT('Origin',(-1.5,1.9,1.75));
#7939=CARTESIAN_POINT('',(-1.43596875762567,1.7,1.7));
#7940=CARTESIAN_POINT('Origin',(-1.5,-1.9,1.7));
#7941=CARTESIAN_POINT('',(-1.43596875762567,-1.7,1.7));
#7942=CARTESIAN_POINT('',(-1.56403124237433,-1.7,1.7));
#7943=CARTESIAN_POINT('',(-0.75,-1.7,1.7));
#7944=CARTESIAN_POINT('Origin',(-1.5,-1.9,1.7));
#7945=CARTESIAN_POINT('Origin',(-1.5,-1.9,1.7));
#7946=CARTESIAN_POINT('',(-1.43596875762567,-1.7,1.75));
#7947=CARTESIAN_POINT('',(-1.43596875762567,-1.7,1.7));
#7948=CARTESIAN_POINT('',(-1.71,-1.9,1.75));
#7949=CARTESIAN_POINT('Origin',(-1.5,-1.9,1.75));
#7950=CARTESIAN_POINT('',(-1.71,-1.9,2.4));
#7951=CARTESIAN_POINT('',(-1.71,-1.9,1.7));
#7952=CARTESIAN_POINT('Origin',(-1.5,-1.9,2.4));
#7953=CARTESIAN_POINT('',(-1.56403124237433,-1.7,1.75));
#7954=CARTESIAN_POINT('Origin',(-1.5,-1.9,1.75));
#7955=CARTESIAN_POINT('',(-1.56403124237433,-1.7,1.7));
#7956=CARTESIAN_POINT('Origin',(1.5,1.9,1.7));
#7957=CARTESIAN_POINT('',(1.43596875762567,1.7,1.7));
#7958=CARTESIAN_POINT('',(1.56403124237433,1.7,1.7));
#7959=CARTESIAN_POINT('',(0.75,1.7,1.7));
#7960=CARTESIAN_POINT('Origin',(1.5,1.9,1.7));
#7961=CARTESIAN_POINT('Origin',(1.5,1.9,1.7));
#7962=CARTESIAN_POINT('',(1.43596875762567,1.7,1.75));
#7963=CARTESIAN_POINT('',(1.43596875762567,1.7,1.7));
#7964=CARTESIAN_POINT('',(1.29,1.9,1.75));
#7965=CARTESIAN_POINT('Origin',(1.5,1.9,1.75));
#7966=CARTESIAN_POINT('',(1.29,1.9,2.4));
#7967=CARTESIAN_POINT('',(1.29,1.9,1.7));
#7968=CARTESIAN_POINT('Origin',(1.5,1.9,2.4));
#7969=CARTESIAN_POINT('',(1.56403124237433,1.7,1.75));
#7970=CARTESIAN_POINT('Origin',(1.5,1.9,1.75));
#7971=CARTESIAN_POINT('',(1.56403124237433,1.7,1.7));
#7972=CARTESIAN_POINT('Origin',(0.,-1.7,1.75));
#7973=CARTESIAN_POINT('',(0.,-1.7,1.75));
#7974=CARTESIAN_POINT('',(-1.97,-1.7,1.75));
#7975=CARTESIAN_POINT('',(0.,-1.7,1.75));
#7976=CARTESIAN_POINT('',(-1.97,-1.7,0.43));
#7977=CARTESIAN_POINT('',(-1.97,-1.7,1.75));
#7978=CARTESIAN_POINT('',(1.97,-1.7,0.43));
#7979=CARTESIAN_POINT('',(0.,-1.7,0.43));
#7980=CARTESIAN_POINT('',(1.97,-1.7,1.75));
#7981=CARTESIAN_POINT('',(1.97,-1.7,1.75));
#7982=CARTESIAN_POINT('',(0.,-1.7,1.75));
#7983=CARTESIAN_POINT('Origin',(0.,1.7,0.43));
#7984=CARTESIAN_POINT('',(0.,1.7,1.75));
#7985=CARTESIAN_POINT('',(1.97,1.7,1.75));
#7986=CARTESIAN_POINT('',(0.,1.7,1.75));
#7987=CARTESIAN_POINT('',(1.97,1.7,0.43));
#7988=CARTESIAN_POINT('',(1.97,1.7,0.43));
#7989=CARTESIAN_POINT('',(-1.97,1.7,0.43));
#7990=CARTESIAN_POINT('',(0.,1.7,0.43));
#7991=CARTESIAN_POINT('',(-1.97,1.7,1.75));
#7992=CARTESIAN_POINT('',(-1.97,1.7,0.43));
#7993=CARTESIAN_POINT('',(0.,1.7,1.75));
#7994=CARTESIAN_POINT('Origin',(-1.97,0.,1.415));
#7995=CARTESIAN_POINT('',(-1.97,-2.35,1.75));
#7996=CARTESIAN_POINT('',(-1.97,-2.35,1.75));
#7997=CARTESIAN_POINT('',(-1.97,-2.35,2.4));
#7998=CARTESIAN_POINT('',(-1.97,-2.35,2.4));
#7999=CARTESIAN_POINT('',(-1.97,2.35,2.4));
#8000=CARTESIAN_POINT('',(-1.97,2.35,2.4));
#8001=CARTESIAN_POINT('',(-1.97,2.35,1.75));
#8002=CARTESIAN_POINT('',(-1.97,2.35,1.75));
#8003=CARTESIAN_POINT('',(-1.97,1.7,1.75));
#8004=CARTESIAN_POINT('',(-1.97,0.78,0.43));
#8005=CARTESIAN_POINT('',(-1.97,0.78,0.43));
#8006=CARTESIAN_POINT('',(-1.97,0.78,1.55));
#8007=CARTESIAN_POINT('',(-1.97,0.78,1.55));
#8008=CARTESIAN_POINT('',(-1.97,-0.78,1.55));
#8009=CARTESIAN_POINT('',(-1.97,-0.78,1.55));
#8010=CARTESIAN_POINT('',(-1.97,-0.78,0.43));
#8011=CARTESIAN_POINT('',(-1.97,-0.78,0.43));
#8012=CARTESIAN_POINT('',(-1.97,-1.7,0.43));
#8013=CARTESIAN_POINT('Origin',(0.,-2.35,1.75));
#8014=CARTESIAN_POINT('',(1.97,-2.35,1.75));
#8015=CARTESIAN_POINT('',(1.97,-2.35,1.75));
#8016=CARTESIAN_POINT('',(0.,-2.35,1.75));
#8017=CARTESIAN_POINT('Origin',(0.,-2.35,2.4));
#8018=CARTESIAN_POINT('',(1.97,-2.35,2.4));
#8019=CARTESIAN_POINT('',(1.97,-2.35,2.4));
#8020=CARTESIAN_POINT('',(0.,-2.35,2.4));
#8021=CARTESIAN_POINT('Origin',(0.,2.35,2.4));
#8022=CARTESIAN_POINT('',(1.97,2.35,2.4));
#8023=CARTESIAN_POINT('',(1.97,2.35,2.4));
#8024=CARTESIAN_POINT('',(0.,2.35,2.4));
#8025=CARTESIAN_POINT('Origin',(0.,2.35,1.75));
#8026=CARTESIAN_POINT('',(1.97,2.35,1.75));
#8027=CARTESIAN_POINT('',(1.97,2.35,1.75));
#8028=CARTESIAN_POINT('',(0.,2.35,1.75));
#8029=CARTESIAN_POINT('Origin',(0.,1.7,1.75));
#8030=CARTESIAN_POINT('',(1.97,1.7,1.75));
#8031=CARTESIAN_POINT('Origin',(0.,0.78,0.43));
#8032=CARTESIAN_POINT('',(1.97,0.78,0.43));
#8033=CARTESIAN_POINT('',(1.97,0.78,0.43));
#8034=CARTESIAN_POINT('',(0.,0.78,0.43));
#8035=CARTESIAN_POINT('Origin',(0.,0.78,1.55));
#8036=CARTESIAN_POINT('',(1.97,0.78,1.55));
#8037=CARTESIAN_POINT('',(1.97,0.78,1.55));
#8038=CARTESIAN_POINT('',(0.,0.78,1.55));
#8039=CARTESIAN_POINT('Origin',(0.,-0.78,1.55));
#8040=CARTESIAN_POINT('',(1.97,-0.78,1.55));
#8041=CARTESIAN_POINT('',(1.97,-0.78,1.55));
#8042=CARTESIAN_POINT('',(0.,-0.78,1.55));
#8043=CARTESIAN_POINT('Origin',(0.,-0.78,0.43));
#8044=CARTESIAN_POINT('',(1.97,-0.78,0.43));
#8045=CARTESIAN_POINT('',(1.97,-0.78,0.43));
#8046=CARTESIAN_POINT('',(0.,-0.78,0.43));
#8047=CARTESIAN_POINT('Origin',(0.,-1.7,0.43));
#8048=CARTESIAN_POINT('',(1.97,-1.7,0.43));
#8049=CARTESIAN_POINT('Origin',(1.97,0.,1.415));
#8467=UNCERTAINTY_MEASURE_WITH_UNIT(LENGTH_MEASURE(0.001),#8500,
'DISTANCE_ACCURACY_VALUE',
'Maximum model space distance between geometric entities at asserted c
onnectivities');
#8476=UNCERTAINTY_MEASURE_WITH_UNIT(LENGTH_MEASURE(0.001),#8500,
'DISTANCE_ACCURACY_VALUE',
'Maximum model space distance between geometric entities at asserted c
onnectivities');
#8490=(
GEOMETRIC_REPRESENTATION_CONTEXT(3)
GLOBAL_UNCERTAINTY_ASSIGNED_CONTEXT((#8467))
GLOBAL_UNIT_ASSIGNED_CONTEXT((#8500,#8502,#8503))
REPRESENTATION_CONTEXT('','3D')
);
#8499=(
GEOMETRIC_REPRESENTATION_CONTEXT(3)
GLOBAL_UNCERTAINTY_ASSIGNED_CONTEXT((#8476))
GLOBAL_UNIT_ASSIGNED_CONTEXT((#8500,#8502,#8503))
REPRESENTATION_CONTEXT('','3D')
);
#8500=(
LENGTH_UNIT()
NAMED_UNIT(*)
SI_UNIT(.CENTI.,.METRE.)
);
#8502=(
NAMED_UNIT(*)
PLANE_ANGLE_UNIT()
SI_UNIT($,.RADIAN.)
);
#8503=(
NAMED_UNIT(*)
SI_UNIT($,.STERADIAN.)
SOLID_ANGLE_UNIT()
);
#8517=SHAPE_DEFINITION_REPRESENTATION(#8539,#8611);
#8539=PRODUCT_DEFINITION_SHAPE('',$,#8634);
#8611=SHAPE_REPRESENTATION('',(#5414),#8490);
#8620=PRODUCT_DEFINITION_CONTEXT('part definition',#8688,'design');
#8634=PRODUCT_DEFINITION('Block','Block',#8656,#8620);
#8656=PRODUCT_DEFINITION_FORMATION('',$,#8703);
#8688=APPLICATION_CONTEXT(
'Core Data for Automotive Mechanical Design Process');
#8689=PRODUCT_CONTEXT('part definition',#8688,'mechanical');
#8703=PRODUCT('Block','Block','Block',(#8689));
#8761=COLOUR_RGB('Dark Blue',0.08,0.2,0.34);
#8762=FILL_AREA_STYLE_COLOUR('',#8761);
#8763=FILL_AREA_STYLE('',(#8762));
#8764=SURFACE_STYLE_FILL_AREA(#8763);
#8765=SURFACE_SIDE_STYLE('',(#8764));
#8766=SURFACE_STYLE_USAGE(.BOTH.,#8765);
#8767=PRESENTATION_STYLE_ASSIGNMENT((#8766));
ENDSEC;
END-ISO-10303-21;
